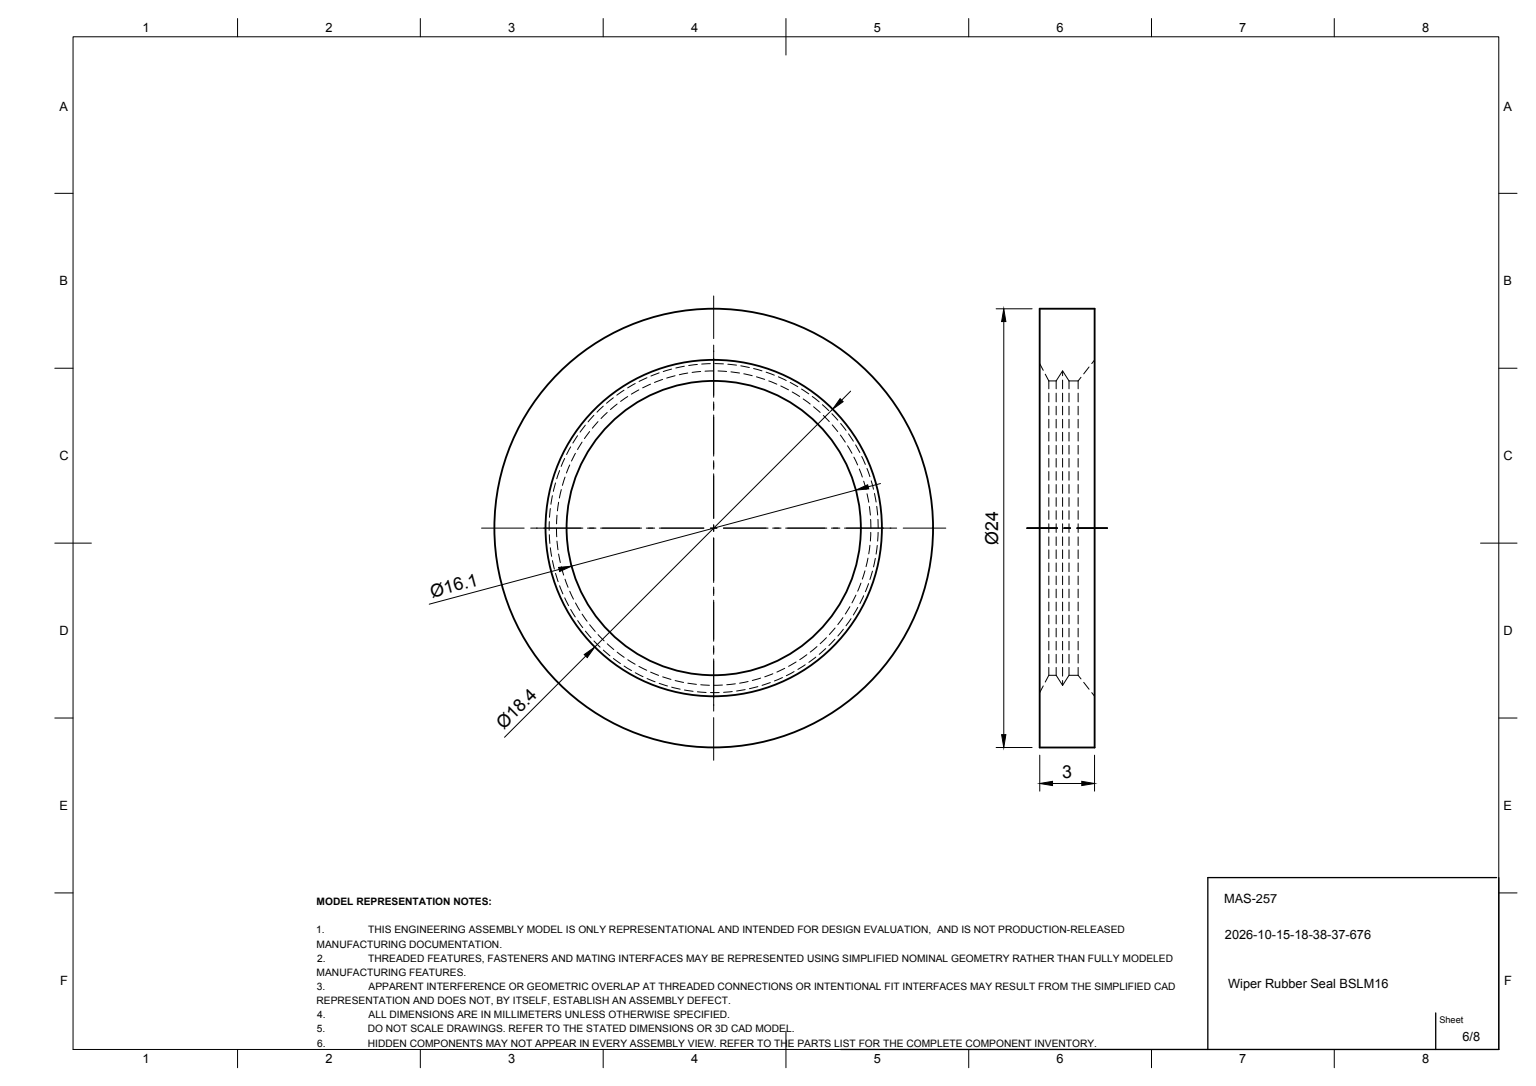
ISO-10303-21;
HEADER;
FILE_DESCRIPTION((''),'2;1');
FILE_NAME('Wiper Rubber Seal BSLM16.step','2026-10-05T22:33:56+05:00',(''),(''),'','','');
FILE_SCHEMA (('AUTOMOTIVE_DESIGN { 1 0 10303 214 3 1 1 }'));
ENDSEC;
DATA;
#10=MECHANICAL_DESIGN_GEOMETRIC_PRESENTATION_REPRESENTATION('',(#434),#16942);
#420=SHAPE_REPRESENTATION_RELATIONSHIP('SRR','None',#17024,#427) ;
#427=ADVANCED_BREP_SHAPE_REPRESENTATION('',(#441),#16940) ;
#434=STYLED_ITEM('',(#17068),#441) ;
#441=MANIFOLD_SOLID_BREP('Wiper Rubber Seal BSLM16',#8183) ;
#731=FACE_BOUND('',#1970,.T.) ;
#732=FACE_BOUND('',#1973,.T.) ;
#967=PLANE('',#8878) ;
#968=PLANE('',#8883) ;
#1054=CYLINDRICAL_SURFACE('',#8881,12.) ;
#1055=CYLINDRICAL_SURFACE('',#8887,8.05) ;
#1056=CYLINDRICAL_SURFACE('',#8893,8.05) ;
#1482=FACE_OUTER_BOUND('',#1969,.T.) ;
#1483=FACE_OUTER_BOUND('',#1971,.T.) ;
#1484=FACE_OUTER_BOUND('',#1972,.T.) ;
#1485=FACE_OUTER_BOUND('',#1974,.T.) ;
#1486=FACE_OUTER_BOUND('',#1975,.T.) ;
#1487=FACE_OUTER_BOUND('',#1976,.T.) ;
#1488=FACE_OUTER_BOUND('',#1977,.T.) ;
#1489=FACE_OUTER_BOUND('',#1978,.T.) ;
#1490=FACE_OUTER_BOUND('',#1979,.T.) ;
#1969=EDGE_LOOP('',(#7615)) ;
#1970=EDGE_LOOP('',(#7616)) ;
#1971=EDGE_LOOP('',(#7617,#7618,#7619,#7620)) ;
#1972=EDGE_LOOP('',(#7621)) ;
#1973=EDGE_LOOP('',(#7622)) ;
#1974=EDGE_LOOP('',(#7623,#7624,#7625,#7626)) ;
#1975=EDGE_LOOP('',(#7627,#7628,#7629,#7630)) ;
#1976=EDGE_LOOP('',(#7631,#7632,#7633,#7634)) ;
#1977=EDGE_LOOP('',(#7635,#7636,#7637,#7638)) ;
#1978=EDGE_LOOP('',(#7639,#7640,#7641,#7642)) ;
#1979=EDGE_LOOP('',(#7643,#7644,#7645,#7646)) ;
#2529=LINE('',#16781,#3091) ;
#2530=LINE('',#16787,#3092) ;
#2531=LINE('',#16791,#3093) ;
#2532=LINE('',#16795,#3094) ;
#2533=LINE('',#16799,#3095) ;
#2534=LINE('',#16803,#3096) ;
#2535=LINE('',#16806,#3097) ;
#3091=VECTOR('',#10745,12.) ;
#3092=VECTOR('',#10752,8.625) ;
#3093=VECTOR('',#10757,8.05) ;
#3094=VECTOR('',#10762,8.325) ;
#3095=VECTOR('',#10767,8.325) ;
#3096=VECTOR('',#10772,8.05) ;
#3097=VECTOR('',#10777,8.525) ;
#3381=CIRCLE('',#8879,12.) ;
#3382=CIRCLE('',#8880,9.) ;
#3383=CIRCLE('',#8882,12.) ;
#3384=CIRCLE('',#8884,9.2) ;
#3385=CIRCLE('',#8886,8.05) ;
#3386=CIRCLE('',#8888,8.05) ;
#3387=CIRCLE('',#8890,8.6) ;
#3388=CIRCLE('',#8892,8.05) ;
#3389=CIRCLE('',#8894,8.05) ;
#4144=VERTEX_POINT('',#16774) ;
#4145=VERTEX_POINT('',#16776) ;
#4146=VERTEX_POINT('',#16779) ;
#4147=VERTEX_POINT('',#16783) ;
#4148=VERTEX_POINT('',#16786) ;
#4149=VERTEX_POINT('',#16790) ;
#4150=VERTEX_POINT('',#16794) ;
#4151=VERTEX_POINT('',#16798) ;
#4152=VERTEX_POINT('',#16802) ;
#5305=EDGE_CURVE('',#4144,#4144,#3381,.T.) ;
#5306=EDGE_CURVE('',#4145,#4145,#3382,.T.) ;
#5307=EDGE_CURVE('',#4146,#4146,#3383,.T.) ;
#5308=EDGE_CURVE('',#4146,#4144,#2529,.T.) ;
#5309=EDGE_CURVE('',#4147,#4147,#3384,.T.) ;
#5310=EDGE_CURVE('',#4147,#4148,#2530,.T.) ;
#5311=EDGE_CURVE('',#4148,#4148,#3385,.T.) ;
#5312=EDGE_CURVE('',#4148,#4149,#2531,.T.) ;
#5313=EDGE_CURVE('',#4149,#4149,#3386,.T.) ;
#5314=EDGE_CURVE('',#4149,#4150,#2532,.T.) ;
#5315=EDGE_CURVE('',#4150,#4150,#3387,.T.) ;
#5316=EDGE_CURVE('',#4150,#4151,#2533,.T.) ;
#5317=EDGE_CURVE('',#4151,#4151,#3388,.T.) ;
#5318=EDGE_CURVE('',#4151,#4152,#2534,.T.) ;
#5319=EDGE_CURVE('',#4152,#4152,#3389,.T.) ;
#5320=EDGE_CURVE('',#4152,#4145,#2535,.T.) ;
#7615=ORIENTED_EDGE('',*,*,#5305,.F.) ;
#7616=ORIENTED_EDGE('',*,*,#5306,.T.) ;
#7617=ORIENTED_EDGE('',*,*,#5307,.F.) ;
#7618=ORIENTED_EDGE('',*,*,#5308,.T.) ;
#7619=ORIENTED_EDGE('',*,*,#5305,.T.) ;
#7620=ORIENTED_EDGE('',*,*,#5308,.F.) ;
#7621=ORIENTED_EDGE('',*,*,#5307,.T.) ;
#7622=ORIENTED_EDGE('',*,*,#5309,.F.) ;
#7623=ORIENTED_EDGE('',*,*,#5309,.T.) ;
#7624=ORIENTED_EDGE('',*,*,#5310,.T.) ;
#7625=ORIENTED_EDGE('',*,*,#5311,.F.) ;
#7626=ORIENTED_EDGE('',*,*,#5310,.F.) ;
#7627=ORIENTED_EDGE('',*,*,#5311,.T.) ;
#7628=ORIENTED_EDGE('',*,*,#5312,.T.) ;
#7629=ORIENTED_EDGE('',*,*,#5313,.F.) ;
#7630=ORIENTED_EDGE('',*,*,#5312,.F.) ;
#7631=ORIENTED_EDGE('',*,*,#5313,.T.) ;
#7632=ORIENTED_EDGE('',*,*,#5314,.T.) ;
#7633=ORIENTED_EDGE('',*,*,#5315,.F.) ;
#7634=ORIENTED_EDGE('',*,*,#5314,.F.) ;
#7635=ORIENTED_EDGE('',*,*,#5315,.T.) ;
#7636=ORIENTED_EDGE('',*,*,#5316,.T.) ;
#7637=ORIENTED_EDGE('',*,*,#5317,.F.) ;
#7638=ORIENTED_EDGE('',*,*,#5316,.F.) ;
#7639=ORIENTED_EDGE('',*,*,#5317,.T.) ;
#7640=ORIENTED_EDGE('',*,*,#5318,.T.) ;
#7641=ORIENTED_EDGE('',*,*,#5319,.F.) ;
#7642=ORIENTED_EDGE('',*,*,#5318,.F.) ;
#7643=ORIENTED_EDGE('',*,*,#5319,.T.) ;
#7644=ORIENTED_EDGE('',*,*,#5320,.T.) ;
#7645=ORIENTED_EDGE('',*,*,#5306,.F.) ;
#7646=ORIENTED_EDGE('',*,*,#5320,.F.) ;
#7732=CONICAL_SURFACE('',#8885,8.625,0.906750163968216) ;
#7733=CONICAL_SURFACE('',#8889,8.325,1.00406710927139) ;
#7734=CONICAL_SURFACE('',#8891,8.325,1.00406710927139) ;
#7735=CONICAL_SURFACE('',#8895,8.525,1.08631839775788) ;
#8157=ADVANCED_FACE('',(#1482,#731),#967,.T.) ;
#8158=ADVANCED_FACE('',(#1483),#1054,.T.) ;
#8159=ADVANCED_FACE('',(#1484,#732),#968,.T.) ;
#8160=ADVANCED_FACE('',(#1485),#7732,.F.) ;
#8161=ADVANCED_FACE('',(#1486),#1055,.F.) ;
#8162=ADVANCED_FACE('',(#1487),#7733,.F.) ;
#8163=ADVANCED_FACE('',(#1488),#7734,.F.) ;
#8164=ADVANCED_FACE('',(#1489),#1056,.F.) ;
#8165=ADVANCED_FACE('',(#1490),#7735,.F.) ;
#8183=CLOSED_SHELL('',(#8157,#8158,#8159,#8160,#8161,#8162,#8163,#8164,
#8165)) ;
#8877=AXIS2_PLACEMENT_3D('',#16772,#10733,#10734) ;
#8878=AXIS2_PLACEMENT_3D('',#16773,#10735,#10736) ;
#8879=AXIS2_PLACEMENT_3D('',#16775,#10737,#10738) ;
#8880=AXIS2_PLACEMENT_3D('',#16777,#10739,#10740) ;
#8881=AXIS2_PLACEMENT_3D('',#16778,#10741,#10742) ;
#8882=AXIS2_PLACEMENT_3D('',#16780,#10743,#10744) ;
#8883=AXIS2_PLACEMENT_3D('',#16782,#10746,#10747) ;
#8884=AXIS2_PLACEMENT_3D('',#16784,#10748,#10749) ;
#8885=AXIS2_PLACEMENT_3D('',#16785,#10750,#10751) ;
#8886=AXIS2_PLACEMENT_3D('',#16788,#10753,#10754) ;
#8887=AXIS2_PLACEMENT_3D('',#16789,#10755,#10756) ;
#8888=AXIS2_PLACEMENT_3D('',#16792,#10758,#10759) ;
#8889=AXIS2_PLACEMENT_3D('',#16793,#10760,#10761) ;
#8890=AXIS2_PLACEMENT_3D('',#16796,#10763,#10764) ;
#8891=AXIS2_PLACEMENT_3D('',#16797,#10765,#10766) ;
#8892=AXIS2_PLACEMENT_3D('',#16800,#10768,#10769) ;
#8893=AXIS2_PLACEMENT_3D('',#16801,#10770,#10771) ;
#8894=AXIS2_PLACEMENT_3D('',#16804,#10773,#10774) ;
#8895=AXIS2_PLACEMENT_3D('',#16805,#10775,#10776) ;
#10733=DIRECTION('axis',(0.,0.,1.)) ;
#10734=DIRECTION('refdir',(1.,0.,0.)) ;
#10735=DIRECTION('center_axis',(-1.,0.,0.)) ;
#10736=DIRECTION('ref_axis',(0.,0.,1.)) ;
#10737=DIRECTION('center_axis',(1.,0.,0.)) ;
#10738=DIRECTION('ref_axis',(0.,0.,-1.)) ;
#10739=DIRECTION('center_axis',(1.,0.,0.)) ;
#10740=DIRECTION('ref_axis',(0.,0.,-1.)) ;
#10741=DIRECTION('center_axis',(1.,0.,0.)) ;
#10742=DIRECTION('ref_axis',(0.,1.,0.)) ;
#10743=DIRECTION('center_axis',(1.,0.,0.)) ;
#10744=DIRECTION('ref_axis',(0.,0.,-1.)) ;
#10745=DIRECTION('',(-1.,0.,0.)) ;
#10746=DIRECTION('center_axis',(1.,0.,0.)) ;
#10747=DIRECTION('ref_axis',(0.,0.,-1.)) ;
#10748=DIRECTION('center_axis',(1.,0.,0.)) ;
#10749=DIRECTION('ref_axis',(0.,0.,-1.)) ;
#10750=DIRECTION('center_axis',(1.,0.,0.)) ;
#10751=DIRECTION('ref_axis',(0.,1.,0.)) ;
#10752=DIRECTION('',(-0.616308261658108,0.787505001007588,9.64415478796476E-17)) ;
#10753=DIRECTION('center_axis',(1.,0.,0.)) ;
#10754=DIRECTION('ref_axis',(0.,0.,-1.)) ;
#10755=DIRECTION('center_axis',(1.,0.,0.)) ;
#10756=DIRECTION('ref_axis',(0.,1.,0.)) ;
#10757=DIRECTION('',(-1.,0.,0.)) ;
#10758=DIRECTION('center_axis',(1.,0.,0.)) ;
#10759=DIRECTION('ref_axis',(0.,0.,-1.)) ;
#10760=DIRECTION('center_axis',(-1.,0.,0.)) ;
#10761=DIRECTION('ref_axis',(0.,1.,0.)) ;
#10762=DIRECTION('',(-0.536875492193157,-0.843661487732109,-1.03318734051502E-16)) ;
#10763=DIRECTION('center_axis',(1.,0.,0.)) ;
#10764=DIRECTION('ref_axis',(0.,0.,-1.)) ;
#10765=DIRECTION('center_axis',(1.,0.,0.)) ;
#10766=DIRECTION('ref_axis',(0.,1.,0.)) ;
#10767=DIRECTION('',(-0.536875492193157,0.843661487732109,1.03318734051502E-16)) ;
#10768=DIRECTION('center_axis',(1.,0.,0.)) ;
#10769=DIRECTION('ref_axis',(0.,0.,-1.)) ;
#10770=DIRECTION('center_axis',(1.,0.,0.)) ;
#10771=DIRECTION('ref_axis',(0.,1.,0.)) ;
#10772=DIRECTION('',(-1.,0.,0.)) ;
#10773=DIRECTION('center_axis',(1.,0.,0.)) ;
#10774=DIRECTION('ref_axis',(0.,0.,-1.)) ;
#10775=DIRECTION('center_axis',(-1.,0.,0.)) ;
#10776=DIRECTION('ref_axis',(0.,1.,0.)) ;
#10777=DIRECTION('',(-0.465746432832619,-0.884918222381984,-1.08371226854726E-16)) ;
#16772=CARTESIAN_POINT('',(0.,0.,0.)) ;
#16773=CARTESIAN_POINT('Origin',(29.1,37.5,25.5)) ;
#16774=CARTESIAN_POINT('',(29.1,13.5,25.5)) ;
#16775=CARTESIAN_POINT('Origin',(29.1,25.5,25.5)) ;
#16776=CARTESIAN_POINT('',(29.1,16.5,25.5)) ;
#16777=CARTESIAN_POINT('Origin',(29.1,25.5,25.5)) ;
#16778=CARTESIAN_POINT('Origin',(30.6,25.5,25.5)) ;
#16779=CARTESIAN_POINT('',(32.1,13.5,25.5)) ;
#16780=CARTESIAN_POINT('Origin',(32.1,25.5,25.5)) ;
#16781=CARTESIAN_POINT('',(30.6,13.5,25.5)) ;
#16782=CARTESIAN_POINT('Origin',(32.1,34.7,25.5)) ;
#16783=CARTESIAN_POINT('',(32.1,16.3,25.5)) ;
#16784=CARTESIAN_POINT('Origin',(32.1,25.5,25.5)) ;
#16785=CARTESIAN_POINT('Origin',(31.65,25.5,25.5)) ;
#16786=CARTESIAN_POINT('',(31.2,17.45,25.5)) ;
#16787=CARTESIAN_POINT('',(31.65,16.875,25.5)) ;
#16788=CARTESIAN_POINT('Origin',(31.2,25.5,25.5)) ;
#16789=CARTESIAN_POINT('Origin',(30.95,25.5,25.5)) ;
#16790=CARTESIAN_POINT('',(30.7,17.45,25.5)) ;
#16791=CARTESIAN_POINT('',(30.95,17.45,25.5)) ;
#16792=CARTESIAN_POINT('Origin',(30.7,25.5,25.5)) ;
#16793=CARTESIAN_POINT('Origin',(30.525,25.5,25.5)) ;
#16794=CARTESIAN_POINT('',(30.35,16.9,25.5)) ;
#16795=CARTESIAN_POINT('',(30.525,17.175,25.5)) ;
#16796=CARTESIAN_POINT('Origin',(30.35,25.5,25.5)) ;
#16797=CARTESIAN_POINT('Origin',(30.175,25.5,25.5)) ;
#16798=CARTESIAN_POINT('',(30.,17.45,25.5)) ;
#16799=CARTESIAN_POINT('',(30.175,17.175,25.5)) ;
#16800=CARTESIAN_POINT('Origin',(30.,25.5,25.5)) ;
#16801=CARTESIAN_POINT('Origin',(29.8,25.5,25.5)) ;
#16802=CARTESIAN_POINT('',(29.6,17.45,25.5)) ;
#16803=CARTESIAN_POINT('',(29.8,17.45,25.5)) ;
#16804=CARTESIAN_POINT('Origin',(29.6,25.5,25.5)) ;
#16805=CARTESIAN_POINT('Origin',(29.35,25.5,25.5)) ;
#16806=CARTESIAN_POINT('',(29.35,16.975,25.5)) ;
#16931=UNCERTAINTY_MEASURE_WITH_UNIT(LENGTH_MEASURE(0.01),#16943,
'DISTANCE_ACCURACY_VALUE',
'Maximum model space distance between geometric entities at asserted c
onnectivities') ;
#16933=UNCERTAINTY_MEASURE_WITH_UNIT(LENGTH_MEASURE(0.01),#16943,
'DISTANCE_ACCURACY_VALUE',
'Maximum model space distance between geometric entities at asserted c
onnectivities') ;
#16940=(
GEOMETRIC_REPRESENTATION_CONTEXT(3)
GLOBAL_UNCERTAINTY_ASSIGNED_CONTEXT((#16931))
GLOBAL_UNIT_ASSIGNED_CONTEXT((#16943,#16945,#16946))
REPRESENTATION_CONTEXT('','3D')
) ;
#16942=(
GEOMETRIC_REPRESENTATION_CONTEXT(3)
GLOBAL_UNCERTAINTY_ASSIGNED_CONTEXT((#16933))
GLOBAL_UNIT_ASSIGNED_CONTEXT((#16943,#16945,#16946))
REPRESENTATION_CONTEXT('','3D')
) ;
#16943=(
LENGTH_UNIT()
NAMED_UNIT(*)
SI_UNIT(.MILLI.,.METRE.)
) ;
#16945=(
NAMED_UNIT(*)
PLANE_ANGLE_UNIT()
SI_UNIT($,.RADIAN.)
) ;
#16946=(
NAMED_UNIT(*)
SI_UNIT($,.STERADIAN.)
SOLID_ANGLE_UNIT()
) ;
#16953=SHAPE_DEFINITION_REPRESENTATION(#16961,#17024) ;
#16961=PRODUCT_DEFINITION_SHAPE('',$,#17033) ;
#17024=SHAPE_REPRESENTATION('',(#8877),#16940) ;
#17026=PRODUCT_DEFINITION_CONTEXT('part definition',#17052,'design') ;
#17033=PRODUCT_DEFINITION('Wiper Rubber Seal BSLM16',
'Wiper Rubber Seal BSLM16',#17041,#17026) ;
#17041=PRODUCT_DEFINITION_FORMATION('',$,#17060) ;
#17052=APPLICATION_CONTEXT(
'Core Data for Automotive Mechanical Design Process') ;
#17053=PRODUCT_CONTEXT('part definition',#17052,'mechanical') ;
#17060=PRODUCT('Wiper Rubber Seal BSLM16','Wiper Rubber Seal BSLM16',$,(#17053)) ;
#17068=PRESENTATION_STYLE_ASSIGNMENT((#17076)) ;
#17076=SURFACE_STYLE_USAGE(.BOTH.,#17084) ;
#17084=SURFACE_SIDE_STYLE('',(#17092)) ;
#17092=SURFACE_STYLE_FILL_AREA(#17100) ;
#17100=FILL_AREA_STYLE('Rubber - Soft',(#17108)) ;
#17108=FILL_AREA_STYLE_COLOUR('Rubber - Soft',#17116) ;
#17116=COLOUR_RGB('Rubber - Soft', 0.09019608, 0.27058824, 0.51372549) ;
ENDSEC;
END-ISO-10303-21;
